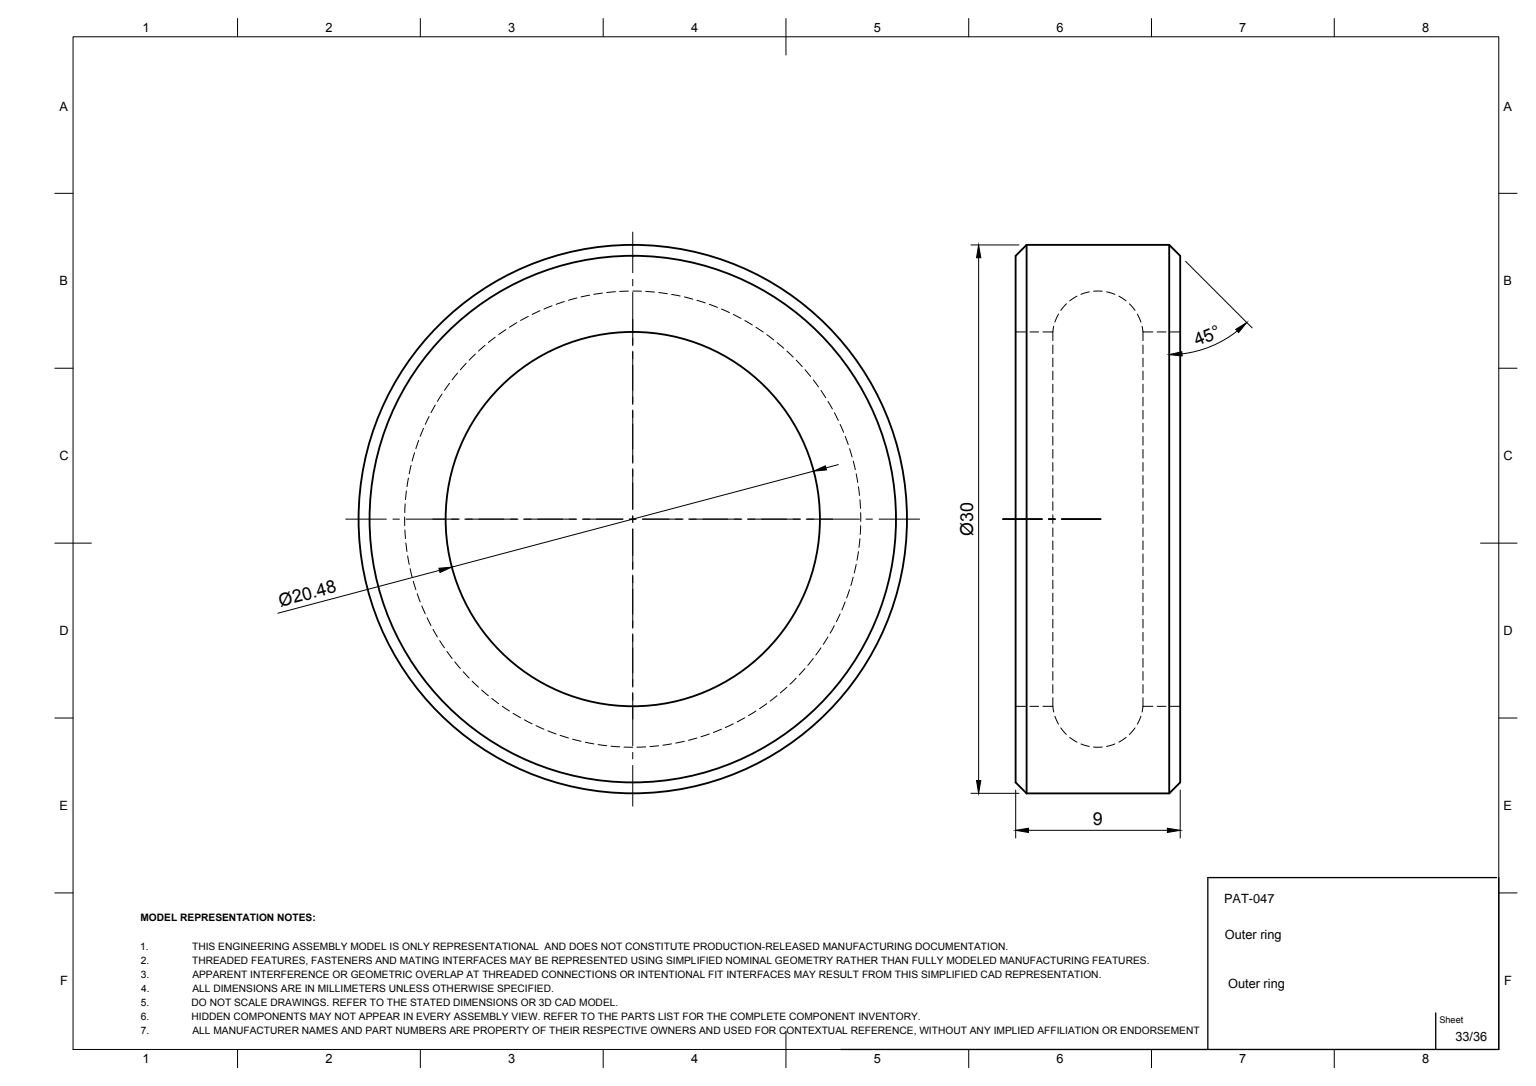
ISO-10303-21;
HEADER;
/* Generated by software containing ST-Developer
 * from STEP Tools, Inc. (www.steptools.com) 
 */

FILE_DESCRIPTION(
/* description */ ('Gravity roller conveyor section'),
/* implementation_level */ '2;1');

FILE_NAME(
/* name */ 'Outer ring.step',
/* time_stamp */ '2026-11-02T07:43:02-08:00',
/* author */ (''),
/* organization */ (''),
/* preprocessor_version */ 'ST-DEVELOPER v20.2',
/* originating_system */ 'Autodesk Translation Framework v15.17.0.0',
/* authorisation */ '');

FILE_SCHEMA (('AUTOMOTIVE_DESIGN { 1 0 10303 214 3 1 1 }'));
ENDSEC;

DATA;
#10=MECHANICAL_DESIGN_GEOMETRIC_PRESENTATION_REPRESENTATION('',(#553),#13821);
#406=TOROIDAL_SURFACE('',#8505,1.,0.247676);
#417=CONICAL_SURFACE('',#8516,1.47,0.785398163397449);
#418=CONICAL_SURFACE('',#8520,1.47,0.785398163397449);
#485=SHAPE_REPRESENTATION_RELATIONSHIP('SRR','None',#14024,#519);
#519=ADVANCED_BREP_SHAPE_REPRESENTATION('',(#593),#13811);
#553=STYLED_ITEM('',(#14191),#593);
#593=MANIFOLD_SOLID_BREP('Body1',#7653);
#680=FACE_BOUND('',#1809,.T.);
#681=FACE_BOUND('',#1814,.T.);
#945=PLANE('',#8513);
#946=PLANE('',#8522);
#1316=FACE_OUTER_BOUND('',#1806,.T.);
#1317=FACE_OUTER_BOUND('',#1807,.T.);
#1318=FACE_OUTER_BOUND('',#1808,.T.);
#1319=FACE_OUTER_BOUND('',#1810,.T.);
#1320=FACE_OUTER_BOUND('',#1811,.T.);
#1321=FACE_OUTER_BOUND('',#1812,.T.);
#1322=FACE_OUTER_BOUND('',#1813,.T.);
#1323=FACE_OUTER_BOUND('',#1815,.T.);
#1806=EDGE_LOOP('',(#6674,#6675,#6676,#6677,#6678,#6679));
#1807=EDGE_LOOP('',(#6680,#6681,#6682,#6683,#6684));
#1808=EDGE_LOOP('',(#6685));
#1809=EDGE_LOOP('',(#6686));
#1810=EDGE_LOOP('',(#6687,#6688,#6689,#6690));
#1811=EDGE_LOOP('',(#6691,#6692,#6693,#6694));
#1812=EDGE_LOOP('',(#6695,#6696,#6697,#6698));
#1813=EDGE_LOOP('',(#6699));
#1814=EDGE_LOOP('',(#6700));
#1815=EDGE_LOOP('',(#6701,#6702,#6703,#6704,#6705));
#2545=LINE('',#12818,#3263);
#2546=LINE('',#12827,#3264);
#2547=LINE('',#12831,#3265);
#2548=LINE('',#12835,#3266);
#2549=LINE('',#12838,#3267);
#3263=VECTOR('',#10354,1.023815);
#3264=VECTOR('',#10365,1.47);
#3265=VECTOR('',#10370,1.5);
#3266=VECTOR('',#10375,1.47);
#3267=VECTOR('',#10380,1.023815);
#3493=CIRCLE('',#8506,1.023815);
#3494=CIRCLE('',#8507,1.023815);
#3495=CIRCLE('',#8508,0.247676);
#3496=CIRCLE('',#8509,1.023815);
#3497=CIRCLE('',#8510,1.023815);
#3498=CIRCLE('',#8512,1.023815);
#3499=CIRCLE('',#8514,1.44);
#3500=CIRCLE('',#8515,1.023815);
#3501=CIRCLE('',#8517,1.5);
#3502=CIRCLE('',#8519,1.5);
#3503=CIRCLE('',#8521,1.44);
#4078=VERTEX_POINT('',#12806);
#4079=VERTEX_POINT('',#12807);
#4080=VERTEX_POINT('',#12810);
#4081=VERTEX_POINT('',#12812);
#4082=VERTEX_POINT('',#12816);
#4083=VERTEX_POINT('',#12820);
#4084=VERTEX_POINT('',#12822);
#4085=VERTEX_POINT('',#12825);
#4086=VERTEX_POINT('',#12829);
#4087=VERTEX_POINT('',#12833);
#4974=EDGE_CURVE('',#4078,#4079,#3493,.T.);
#4975=EDGE_CURVE('',#4079,#4078,#3494,.T.);
#4976=EDGE_CURVE('',#4079,#4080,#3495,.T.);
#4977=EDGE_CURVE('',#4081,#4080,#3496,.T.);
#4978=EDGE_CURVE('',#4080,#4081,#3497,.T.);
#4979=EDGE_CURVE('',#4082,#4082,#3498,.T.);
#4980=EDGE_CURVE('',#4082,#4081,#2545,.T.);
#4981=EDGE_CURVE('',#4083,#4083,#3499,.T.);
#4982=EDGE_CURVE('',#4084,#4084,#3500,.T.);
#4983=EDGE_CURVE('',#4085,#4085,#3501,.T.);
#4984=EDGE_CURVE('',#4085,#4083,#2546,.T.);
#4985=EDGE_CURVE('',#4086,#4086,#3502,.T.);
#4986=EDGE_CURVE('',#4086,#4085,#2547,.T.);
#4987=EDGE_CURVE('',#4087,#4087,#3503,.T.);
#4988=EDGE_CURVE('',#4087,#4086,#2548,.T.);
#4989=EDGE_CURVE('',#4078,#4084,#2549,.T.);
#6674=ORIENTED_EDGE('',*,*,#4974,.F.);
#6675=ORIENTED_EDGE('',*,*,#4975,.F.);
#6676=ORIENTED_EDGE('',*,*,#4976,.T.);
#6677=ORIENTED_EDGE('',*,*,#4977,.F.);
#6678=ORIENTED_EDGE('',*,*,#4978,.F.);
#6679=ORIENTED_EDGE('',*,*,#4976,.F.);
#6680=ORIENTED_EDGE('',*,*,#4979,.T.);
#6681=ORIENTED_EDGE('',*,*,#4980,.T.);
#6682=ORIENTED_EDGE('',*,*,#4977,.T.);
#6683=ORIENTED_EDGE('',*,*,#4978,.T.);
#6684=ORIENTED_EDGE('',*,*,#4980,.F.);
#6685=ORIENTED_EDGE('',*,*,#4981,.F.);
#6686=ORIENTED_EDGE('',*,*,#4982,.T.);
#6687=ORIENTED_EDGE('',*,*,#4983,.F.);
#6688=ORIENTED_EDGE('',*,*,#4984,.T.);
#6689=ORIENTED_EDGE('',*,*,#4981,.T.);
#6690=ORIENTED_EDGE('',*,*,#4984,.F.);
#6691=ORIENTED_EDGE('',*,*,#4985,.F.);
#6692=ORIENTED_EDGE('',*,*,#4986,.T.);
#6693=ORIENTED_EDGE('',*,*,#4983,.T.);
#6694=ORIENTED_EDGE('',*,*,#4986,.F.);
#6695=ORIENTED_EDGE('',*,*,#4987,.F.);
#6696=ORIENTED_EDGE('',*,*,#4988,.T.);
#6697=ORIENTED_EDGE('',*,*,#4985,.T.);
#6698=ORIENTED_EDGE('',*,*,#4988,.F.);
#6699=ORIENTED_EDGE('',*,*,#4987,.T.);
#6700=ORIENTED_EDGE('',*,*,#4979,.F.);
#6701=ORIENTED_EDGE('',*,*,#4974,.T.);
#6702=ORIENTED_EDGE('',*,*,#4975,.T.);
#6703=ORIENTED_EDGE('',*,*,#4989,.T.);
#6704=ORIENTED_EDGE('',*,*,#4982,.F.);
#6705=ORIENTED_EDGE('',*,*,#4989,.F.);
#7185=CYLINDRICAL_SURFACE('',#8511,1.023815);
#7186=CYLINDRICAL_SURFACE('',#8518,1.5);
#7187=CYLINDRICAL_SURFACE('',#8523,1.023815);
#7517=ADVANCED_FACE('',(#1316),#406,.F.);
#7518=ADVANCED_FACE('',(#1317),#7185,.F.);
#7519=ADVANCED_FACE('',(#1318,#680),#945,.T.);
#7520=ADVANCED_FACE('',(#1319),#417,.T.);
#7521=ADVANCED_FACE('',(#1320),#7186,.T.);
#7522=ADVANCED_FACE('',(#1321),#418,.T.);
#7523=ADVANCED_FACE('',(#1322,#681),#946,.T.);
#7524=ADVANCED_FACE('',(#1323),#7187,.F.);
#7653=CLOSED_SHELL('',(#7517,#7518,#7519,#7520,#7521,#7522,#7523,#7524));
#8504=AXIS2_PLACEMENT_3D('',#12804,#10336,#10337);
#8505=AXIS2_PLACEMENT_3D('',#12805,#10338,#10339);
#8506=AXIS2_PLACEMENT_3D('',#12808,#10340,#10341);
#8507=AXIS2_PLACEMENT_3D('',#12809,#10342,#10343);
#8508=AXIS2_PLACEMENT_3D('',#12811,#10344,#10345);
#8509=AXIS2_PLACEMENT_3D('',#12813,#10346,#10347);
#8510=AXIS2_PLACEMENT_3D('',#12814,#10348,#10349);
#8511=AXIS2_PLACEMENT_3D('',#12815,#10350,#10351);
#8512=AXIS2_PLACEMENT_3D('',#12817,#10352,#10353);
#8513=AXIS2_PLACEMENT_3D('',#12819,#10355,#10356);
#8514=AXIS2_PLACEMENT_3D('',#12821,#10357,#10358);
#8515=AXIS2_PLACEMENT_3D('',#12823,#10359,#10360);
#8516=AXIS2_PLACEMENT_3D('',#12824,#10361,#10362);
#8517=AXIS2_PLACEMENT_3D('',#12826,#10363,#10364);
#8518=AXIS2_PLACEMENT_3D('',#12828,#10366,#10367);
#8519=AXIS2_PLACEMENT_3D('',#12830,#10368,#10369);
#8520=AXIS2_PLACEMENT_3D('',#12832,#10371,#10372);
#8521=AXIS2_PLACEMENT_3D('',#12834,#10373,#10374);
#8522=AXIS2_PLACEMENT_3D('',#12836,#10376,#10377);
#8523=AXIS2_PLACEMENT_3D('',#12837,#10378,#10379);
#10336=DIRECTION('axis',(0.,0.,1.));
#10337=DIRECTION('refdir',(1.,0.,0.));
#10338=DIRECTION('center_axis',(0.,-1.,0.));
#10339=DIRECTION('ref_axis',(0.,0.,-1.));
#10340=DIRECTION('center_axis',(0.,-1.,0.));
#10341=DIRECTION('ref_axis',(1.,0.,0.));
#10342=DIRECTION('center_axis',(0.,-1.,0.));
#10343=DIRECTION('ref_axis',(1.,0.,0.));
#10344=DIRECTION('center_axis',(1.,0.,1.22464679914735E-16));
#10345=DIRECTION('ref_axis',(-1.22464679914735E-16,0.,1.));
#10346=DIRECTION('center_axis',(0.,1.,0.));
#10347=DIRECTION('ref_axis',(1.,0.,0.));
#10348=DIRECTION('center_axis',(0.,1.,0.));
#10349=DIRECTION('ref_axis',(1.,0.,0.));
#10350=DIRECTION('center_axis',(0.,-1.,0.));
#10351=DIRECTION('ref_axis',(1.,0.,0.));
#10352=DIRECTION('center_axis',(0.,-1.,0.));
#10353=DIRECTION('ref_axis',(1.,0.,0.));
#10354=DIRECTION('',(0.,1.,0.));
#10355=DIRECTION('center_axis',(0.,1.,0.));
#10356=DIRECTION('ref_axis',(0.,0.,1.));
#10357=DIRECTION('center_axis',(0.,-1.,0.));
#10358=DIRECTION('ref_axis',(1.,0.,0.));
#10359=DIRECTION('center_axis',(0.,-1.,0.));
#10360=DIRECTION('ref_axis',(1.,0.,0.));
#10361=DIRECTION('center_axis',(0.,-1.,0.));
#10362=DIRECTION('ref_axis',(1.,0.,0.));
#10363=DIRECTION('center_axis',(0.,-1.,0.));
#10364=DIRECTION('ref_axis',(1.,0.,0.));
#10365=DIRECTION('',(0.707106781186548,0.707106781186547,8.65956056235494E-17));
#10366=DIRECTION('center_axis',(0.,-1.,0.));
#10367=DIRECTION('ref_axis',(1.,0.,0.));
#10368=DIRECTION('center_axis',(0.,-1.,0.));
#10369=DIRECTION('ref_axis',(1.,0.,0.));
#10370=DIRECTION('',(0.,1.,0.));
#10371=DIRECTION('center_axis',(0.,1.,0.));
#10372=DIRECTION('ref_axis',(1.,0.,0.));
#10373=DIRECTION('center_axis',(0.,-1.,0.));
#10374=DIRECTION('ref_axis',(1.,0.,0.));
#10375=DIRECTION('',(-0.707106781186548,0.707106781186547,-8.65956056235494E-17));
#10376=DIRECTION('center_axis',(0.,-1.,0.));
#10377=DIRECTION('ref_axis',(0.,0.,-1.));
#10378=DIRECTION('center_axis',(0.,-1.,0.));
#10379=DIRECTION('ref_axis',(1.,0.,0.));
#10380=DIRECTION('',(0.,1.,0.));
#12804=CARTESIAN_POINT('',(0.,0.,0.));
#12805=CARTESIAN_POINT('Origin',(0.,0.,0.));
#12806=CARTESIAN_POINT('',(-1.023815,0.246528389340863,-1.25381176266905E-16));
#12807=CARTESIAN_POINT('',(-1.25381176266905E-16,0.246528389340863,1.023815));
#12808=CARTESIAN_POINT('Origin',(0.,0.246528389340863,0.));
#12809=CARTESIAN_POINT('Origin',(0.,0.246528389340863,0.));
#12810=CARTESIAN_POINT('',(-1.25381176266905E-16,-0.246528389340863,1.023815));
#12811=CARTESIAN_POINT('Origin',(-1.22464679914735E-16,0.,1.));
#12812=CARTESIAN_POINT('',(-1.023815,-0.246528389340863,1.25381176266905E-16));
#12813=CARTESIAN_POINT('Origin',(0.,-0.246528389340863,0.));
#12814=CARTESIAN_POINT('Origin',(0.,-0.246528389340863,0.));
#12815=CARTESIAN_POINT('Origin',(0.,0.,0.));
#12816=CARTESIAN_POINT('',(-1.023815,-0.45,-1.25381176266905E-16));
#12817=CARTESIAN_POINT('Origin',(0.,-0.45,0.));
#12818=CARTESIAN_POINT('',(-1.023815,0.,-1.25381176266905E-16));
#12819=CARTESIAN_POINT('Origin',(1.44,0.45,0.));
#12820=CARTESIAN_POINT('',(-1.44,0.45,-1.76349139077219E-16));
#12821=CARTESIAN_POINT('Origin',(0.,0.45,0.));
#12822=CARTESIAN_POINT('',(-1.023815,0.45,-1.25381176266905E-16));
#12823=CARTESIAN_POINT('Origin',(0.,0.45,0.));
#12824=CARTESIAN_POINT('Origin',(0.,0.42,0.));
#12825=CARTESIAN_POINT('',(-1.5,0.39,-1.83697019872103E-16));
#12826=CARTESIAN_POINT('Origin',(0.,0.39,0.));
#12827=CARTESIAN_POINT('',(-1.47,0.42,-1.80023079474661E-16));
#12828=CARTESIAN_POINT('Origin',(0.,0.,0.));
#12829=CARTESIAN_POINT('',(-1.5,-0.39,-1.83697019872103E-16));
#12830=CARTESIAN_POINT('Origin',(0.,-0.39,0.));
#12831=CARTESIAN_POINT('',(-1.5,0.,-1.83697019872103E-16));
#12832=CARTESIAN_POINT('Origin',(0.,-0.42,0.));
#12833=CARTESIAN_POINT('',(-1.44,-0.45,-1.76349139077219E-16));
#12834=CARTESIAN_POINT('Origin',(0.,-0.45,0.));
#12835=CARTESIAN_POINT('',(-1.47,-0.42,-1.80023079474661E-16));
#12836=CARTESIAN_POINT('Origin',(1.023815,-0.45,0.));
#12837=CARTESIAN_POINT('Origin',(0.,0.,0.));
#12838=CARTESIAN_POINT('',(-1.023815,0.,-1.25381176266905E-16));
#13772=UNCERTAINTY_MEASURE_WITH_UNIT(LENGTH_MEASURE(0.001),#13822,
'DISTANCE_ACCURACY_VALUE',
'Maximum model space distance between geometric entities at asserted c
onnectivities');
#13782=UNCERTAINTY_MEASURE_WITH_UNIT(LENGTH_MEASURE(0.001),#13822,
'DISTANCE_ACCURACY_VALUE',
'Maximum model space distance between geometric entities at asserted c
onnectivities');
#13811=(
GEOMETRIC_REPRESENTATION_CONTEXT(3)
GLOBAL_UNCERTAINTY_ASSIGNED_CONTEXT((#13772))
GLOBAL_UNIT_ASSIGNED_CONTEXT((#13822,#13824,#13825))
REPRESENTATION_CONTEXT('','3D')
);
#13821=(
GEOMETRIC_REPRESENTATION_CONTEXT(3)
GLOBAL_UNCERTAINTY_ASSIGNED_CONTEXT((#13782))
GLOBAL_UNIT_ASSIGNED_CONTEXT((#13822,#13824,#13825))
REPRESENTATION_CONTEXT('','3D')
);
#13822=(
LENGTH_UNIT()
NAMED_UNIT(*)
SI_UNIT(.CENTI.,.METRE.)
);
#13824=(
NAMED_UNIT(*)
PLANE_ANGLE_UNIT()
SI_UNIT($,.RADIAN.)
);
#13825=(
NAMED_UNIT(*)
SI_UNIT($,.STERADIAN.)
SOLID_ANGLE_UNIT()
);
#13854=SHAPE_DEFINITION_REPRESENTATION(#13892,#14024);
#13892=PRODUCT_DEFINITION_SHAPE('',$,#14063);
#14024=SHAPE_REPRESENTATION('',(#8504),#13811);
#14034=PRODUCT_DEFINITION_CONTEXT('part definition',#14150,'design');
#14063=PRODUCT_DEFINITION('Outer ring','Outer ring',#14101,#14034);
#14101=PRODUCT_DEFINITION_FORMATION('',$,#14180);
#14150=APPLICATION_CONTEXT(
'Core Data for Automotive Mechanical Design Process');
#14151=PRODUCT_CONTEXT('part definition',#14150,'mechanical');
#14180=PRODUCT('Outer ring','Outer ring','Outer ring',(#14151));
#14191=PRESENTATION_STYLE_ASSIGNMENT((#14196));
#14196=SURFACE_STYLE_USAGE(.BOTH.,#14201);
#14201=SURFACE_SIDE_STYLE('',(#14206));
#14206=SURFACE_STYLE_FILL_AREA(#14211);
#14211=FILL_AREA_STYLE('CAD Library Painted - Steel gray',(#14216));
#14216=FILL_AREA_STYLE_COLOUR('CAD Library Painted - Steel gray',#14221);
#14221=COLOUR_RGB('CAD Library Painted - Steel gray',0.592156862745098,
0.631372549019608,0.67843137254902);
ENDSEC;
END-ISO-10303-21;
